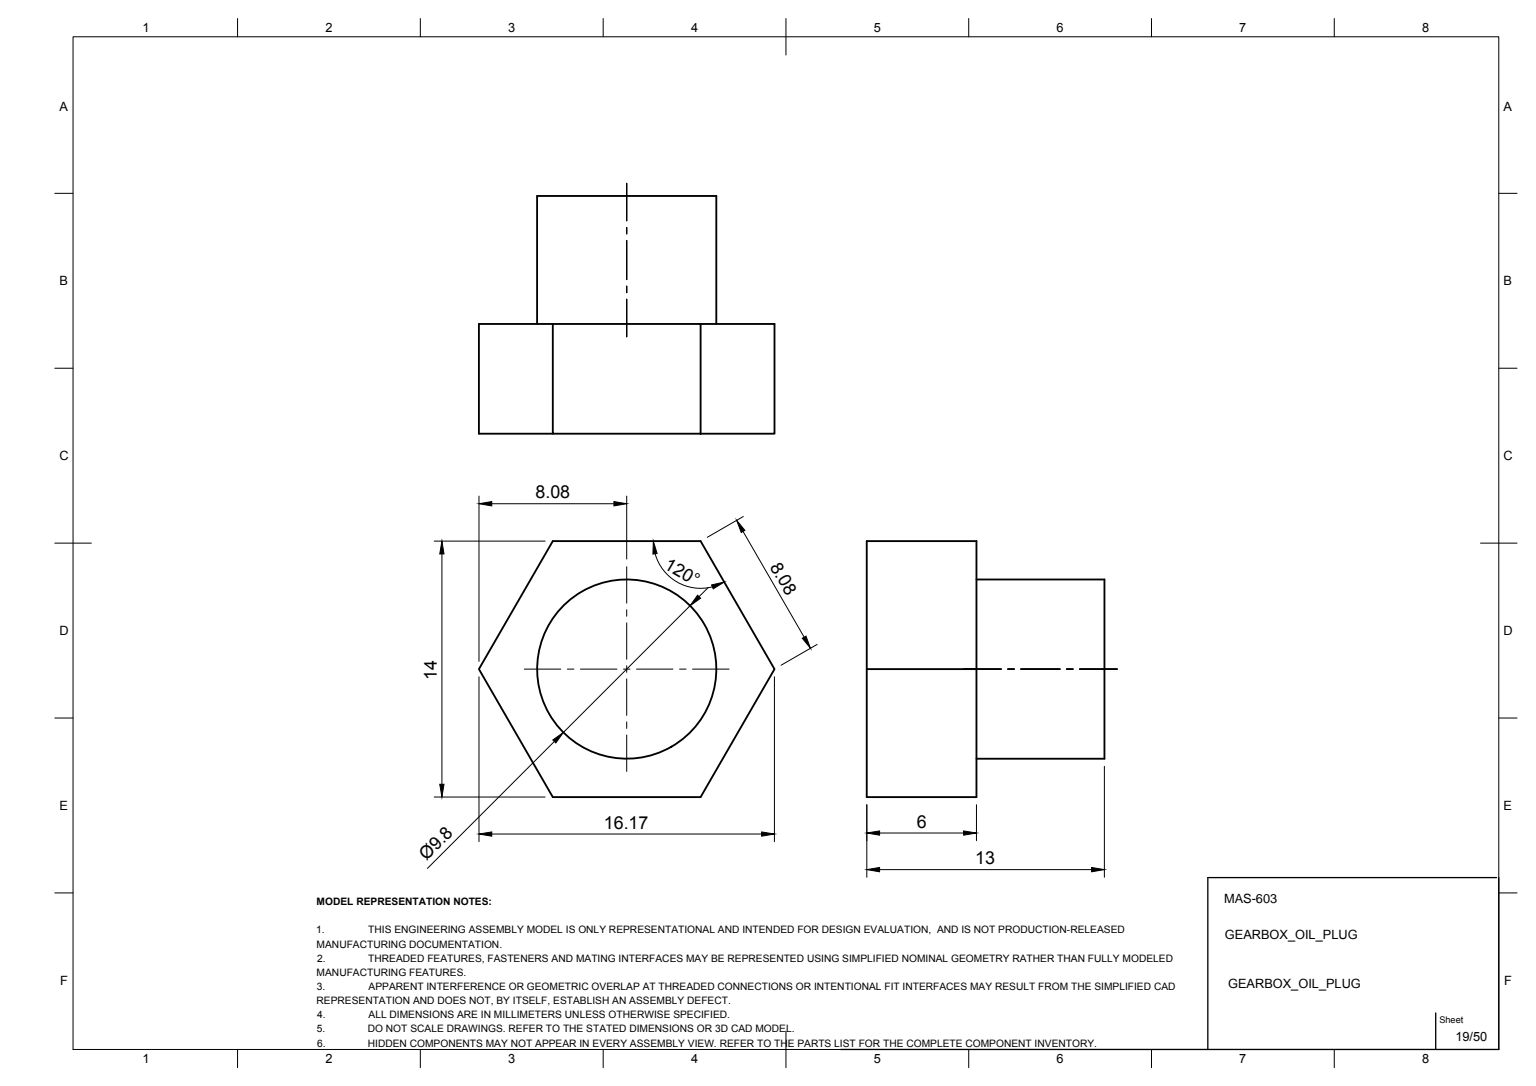
ISO-10303-21;
HEADER;
FILE_DESCRIPTION((''),'2;1');
FILE_NAME('GEARBOX_OIL_PLUG.step','2026-10-01T22:06:14-07:00',(''),(''),'','','');
FILE_SCHEMA (('AUTOMOTIVE_DESIGN { 1 0 10303 214 3 1 1 }'));
ENDSEC;
DATA;
#10=MECHANICAL_DESIGN_GEOMETRIC_PRESENTATION_REPRESENTATION('',(#991),#50440);
#901=SHAPE_REPRESENTATION_RELATIONSHIP('SRR','None',#50633,#946) ;
#946=ADVANCED_BREP_SHAPE_REPRESENTATION('',(#1046),#50402) ;
#991=STYLED_ITEM('',(#50887),#1046) ;
#1046=MANIFOLD_SOLID_BREP('GEARBOX_OIL_PLUG',#28658) ;
#1294=FACE_BOUND('',#4832,.T.) ;
#1979=PLANE('',#30398) ;
#1980=PLANE('',#30399) ;
#1981=PLANE('',#30400) ;
#1982=PLANE('',#30401) ;
#1983=PLANE('',#30402) ;
#1984=PLANE('',#30403) ;
#1985=PLANE('',#30404) ;
#1986=PLANE('',#30405) ;
#1987=PLANE('',#30406) ;
#3091=FACE_OUTER_BOUND('',#4827,.T.) ;
#3092=FACE_OUTER_BOUND('',#4828,.T.) ;
#3093=FACE_OUTER_BOUND('',#4829,.T.) ;
#3094=FACE_OUTER_BOUND('',#4830,.T.) ;
#3095=FACE_OUTER_BOUND('',#4831,.T.) ;
#3096=FACE_OUTER_BOUND('',#4833,.T.) ;
#3097=FACE_OUTER_BOUND('',#4834,.T.) ;
#3098=FACE_OUTER_BOUND('',#4835,.T.) ;
#3099=FACE_OUTER_BOUND('',#4836,.T.) ;
#3100=FACE_OUTER_BOUND('',#4837,.T.) ;
#4827=EDGE_LOOP('',(#22489,#22490,#22491,#22492)) ;
#4828=EDGE_LOOP('',(#22493)) ;
#4829=EDGE_LOOP('',(#22494,#22495,#22496,#22497)) ;
#4830=EDGE_LOOP('',(#22498,#22499,#22500,#22501)) ;
#4831=EDGE_LOOP('',(#22502,#22503,#22504,#22505,#22506,#22507)) ;
#4832=EDGE_LOOP('',(#22508)) ;
#4833=EDGE_LOOP('',(#22509,#22510,#22511,#22512)) ;
#4834=EDGE_LOOP('',(#22513,#22514,#22515,#22516)) ;
#4835=EDGE_LOOP('',(#22517,#22518,#22519,#22520)) ;
#4836=EDGE_LOOP('',(#22521,#22522,#22523,#22524)) ;
#4837=EDGE_LOOP('',(#22525,#22526,#22527,#22528,#22529,#22530)) ;
#7265=LINE('',#45416,#9737) ;
#7266=LINE('',#45422,#9738) ;
#7267=LINE('',#45424,#9739) ;
#7268=LINE('',#45426,#9740) ;
#7269=LINE('',#45427,#9741) ;
#7270=LINE('',#45431,#9742) ;
#7271=LINE('',#45433,#9743) ;
#7272=LINE('',#45435,#9744) ;
#7273=LINE('',#45436,#9745) ;
#7274=LINE('',#45439,#9746) ;
#7275=LINE('',#45440,#9747) ;
#7276=LINE('',#45442,#9748) ;
#7277=LINE('',#45443,#9749) ;
#7278=LINE('',#45446,#9750) ;
#7279=LINE('',#45447,#9751) ;
#7280=LINE('',#45450,#9752) ;
#7281=LINE('',#45451,#9753) ;
#7282=LINE('',#45453,#9754) ;
#7283=LINE('',#45455,#9755) ;
#9737=VECTOR('',#36284,0.49) ;
#9738=VECTOR('',#36291,1.) ;
#9739=VECTOR('',#36292,1.) ;
#9740=VECTOR('',#36293,1.) ;
#9741=VECTOR('',#36294,1.) ;
#9742=VECTOR('',#36297,1.) ;
#9743=VECTOR('',#36298,1.) ;
#9744=VECTOR('',#36299,1.) ;
#9745=VECTOR('',#36300,1.) ;
#9746=VECTOR('',#36303,1.) ;
#9747=VECTOR('',#36304,1.) ;
#9748=VECTOR('',#36305,1.) ;
#9749=VECTOR('',#36306,1.) ;
#9750=VECTOR('',#36309,1.) ;
#9751=VECTOR('',#36310,1.) ;
#9752=VECTOR('',#36313,1.) ;
#9753=VECTOR('',#36314,1.) ;
#9754=VECTOR('',#36317,1.) ;
#9755=VECTOR('',#36320,1.) ;
#11049=CIRCLE('',#30396,0.49) ;
#11050=CIRCLE('',#30397,0.49) ;
#13147=VERTEX_POINT('',#45413) ;
#13148=VERTEX_POINT('',#45415) ;
#13149=VERTEX_POINT('',#45420) ;
#13150=VERTEX_POINT('',#45421) ;
#13151=VERTEX_POINT('',#45423) ;
#13152=VERTEX_POINT('',#45425) ;
#13153=VERTEX_POINT('',#45429) ;
#13154=VERTEX_POINT('',#45430) ;
#13155=VERTEX_POINT('',#45432) ;
#13156=VERTEX_POINT('',#45434) ;
#13157=VERTEX_POINT('',#45438) ;
#13158=VERTEX_POINT('',#45441) ;
#13159=VERTEX_POINT('',#45445) ;
#13160=VERTEX_POINT('',#45449) ;
#16510=EDGE_CURVE('',#13147,#13147,#11049,.T.) ;
#16511=EDGE_CURVE('',#13147,#13148,#7265,.T.) ;
#16512=EDGE_CURVE('',#13148,#13148,#11050,.T.) ;
#16513=EDGE_CURVE('',#13149,#13150,#7266,.T.) ;
#16514=EDGE_CURVE('',#13149,#13151,#7267,.T.) ;
#16515=EDGE_CURVE('',#13152,#13151,#7268,.T.) ;
#16516=EDGE_CURVE('',#13152,#13150,#7269,.T.) ;
#16517=EDGE_CURVE('',#13153,#13154,#7270,.T.) ;
#16518=EDGE_CURVE('',#13153,#13155,#7271,.T.) ;
#16519=EDGE_CURVE('',#13156,#13155,#7272,.T.) ;
#16520=EDGE_CURVE('',#13156,#13154,#7273,.T.) ;
#16521=EDGE_CURVE('',#13157,#13149,#7274,.T.) ;
#16522=EDGE_CURVE('',#13155,#13157,#7275,.T.) ;
#16523=EDGE_CURVE('',#13158,#13153,#7276,.T.) ;
#16524=EDGE_CURVE('',#13151,#13158,#7277,.T.) ;
#16525=EDGE_CURVE('',#13157,#13159,#7278,.T.) ;
#16526=EDGE_CURVE('',#13150,#13159,#7279,.T.) ;
#16527=EDGE_CURVE('',#13158,#13160,#7280,.T.) ;
#16528=EDGE_CURVE('',#13154,#13160,#7281,.T.) ;
#16529=EDGE_CURVE('',#13159,#13156,#7282,.T.) ;
#16530=EDGE_CURVE('',#13160,#13152,#7283,.T.) ;
#22489=ORIENTED_EDGE('',*,*,#16510,.F.) ;
#22490=ORIENTED_EDGE('',*,*,#16511,.T.) ;
#22491=ORIENTED_EDGE('',*,*,#16512,.F.) ;
#22492=ORIENTED_EDGE('',*,*,#16511,.F.) ;
#22493=ORIENTED_EDGE('',*,*,#16512,.T.) ;
#22494=ORIENTED_EDGE('',*,*,#16513,.F.) ;
#22495=ORIENTED_EDGE('',*,*,#16514,.T.) ;
#22496=ORIENTED_EDGE('',*,*,#16515,.F.) ;
#22497=ORIENTED_EDGE('',*,*,#16516,.T.) ;
#22498=ORIENTED_EDGE('',*,*,#16517,.F.) ;
#22499=ORIENTED_EDGE('',*,*,#16518,.T.) ;
#22500=ORIENTED_EDGE('',*,*,#16519,.F.) ;
#22501=ORIENTED_EDGE('',*,*,#16520,.T.) ;
#22502=ORIENTED_EDGE('',*,*,#16514,.F.) ;
#22503=ORIENTED_EDGE('',*,*,#16521,.F.) ;
#22504=ORIENTED_EDGE('',*,*,#16522,.F.) ;
#22505=ORIENTED_EDGE('',*,*,#16518,.F.) ;
#22506=ORIENTED_EDGE('',*,*,#16523,.F.) ;
#22507=ORIENTED_EDGE('',*,*,#16524,.F.) ;
#22508=ORIENTED_EDGE('',*,*,#16510,.T.) ;
#22509=ORIENTED_EDGE('',*,*,#16525,.F.) ;
#22510=ORIENTED_EDGE('',*,*,#16521,.T.) ;
#22511=ORIENTED_EDGE('',*,*,#16513,.T.) ;
#22512=ORIENTED_EDGE('',*,*,#16526,.T.) ;
#22513=ORIENTED_EDGE('',*,*,#16527,.F.) ;
#22514=ORIENTED_EDGE('',*,*,#16523,.T.) ;
#22515=ORIENTED_EDGE('',*,*,#16517,.T.) ;
#22516=ORIENTED_EDGE('',*,*,#16528,.T.) ;
#22517=ORIENTED_EDGE('',*,*,#16519,.T.) ;
#22518=ORIENTED_EDGE('',*,*,#16522,.T.) ;
#22519=ORIENTED_EDGE('',*,*,#16525,.T.) ;
#22520=ORIENTED_EDGE('',*,*,#16529,.T.) ;
#22521=ORIENTED_EDGE('',*,*,#16527,.T.) ;
#22522=ORIENTED_EDGE('',*,*,#16530,.T.) ;
#22523=ORIENTED_EDGE('',*,*,#16515,.T.) ;
#22524=ORIENTED_EDGE('',*,*,#16524,.T.) ;
#22525=ORIENTED_EDGE('',*,*,#16516,.F.) ;
#22526=ORIENTED_EDGE('',*,*,#16530,.F.) ;
#22527=ORIENTED_EDGE('',*,*,#16528,.F.) ;
#22528=ORIENTED_EDGE('',*,*,#16520,.F.) ;
#22529=ORIENTED_EDGE('',*,*,#16529,.F.) ;
#22530=ORIENTED_EDGE('',*,*,#16526,.F.) ;
#26801=CYLINDRICAL_SURFACE('',#30395,0.49) ;
#27826=ADVANCED_FACE('',(#3091),#26801,.T.) ;
#27827=ADVANCED_FACE('',(#3092),#1979,.T.) ;
#27828=ADVANCED_FACE('',(#3093),#1980,.F.) ;
#27829=ADVANCED_FACE('',(#3094),#1981,.F.) ;
#27830=ADVANCED_FACE('',(#3095,#1294),#1982,.T.) ;
#27831=ADVANCED_FACE('',(#3096),#1983,.F.) ;
#27832=ADVANCED_FACE('',(#3097),#1984,.F.) ;
#27833=ADVANCED_FACE('',(#3098),#1985,.F.) ;
#27834=ADVANCED_FACE('',(#3099),#1986,.F.) ;
#27835=ADVANCED_FACE('',(#3100),#1987,.T.) ;
#28658=CLOSED_SHELL('',(#27826,#27827,#27828,#27829,#27830,#27831,#27832,
#27833,#27834,#27835)) ;
#30394=AXIS2_PLACEMENT_3D('',#45411,#36278,#36279) ;
#30395=AXIS2_PLACEMENT_3D('',#45412,#36280,#36281) ;
#30396=AXIS2_PLACEMENT_3D('',#45414,#36282,#36283) ;
#30397=AXIS2_PLACEMENT_3D('',#45417,#36285,#36286) ;
#30398=AXIS2_PLACEMENT_3D('',#45418,#36287,#36288) ;
#30399=AXIS2_PLACEMENT_3D('',#45419,#36289,#36290) ;
#30400=AXIS2_PLACEMENT_3D('',#45428,#36295,#36296) ;
#30401=AXIS2_PLACEMENT_3D('',#45437,#36301,#36302) ;
#30402=AXIS2_PLACEMENT_3D('',#45444,#36307,#36308) ;
#30403=AXIS2_PLACEMENT_3D('',#45448,#36311,#36312) ;
#30404=AXIS2_PLACEMENT_3D('',#45452,#36315,#36316) ;
#30405=AXIS2_PLACEMENT_3D('',#45454,#36318,#36319) ;
#30406=AXIS2_PLACEMENT_3D('',#45456,#36321,#36322) ;
#36278=DIRECTION('axis',(0.,0.,1.)) ;
#36279=DIRECTION('refdir',(1.,0.,0.)) ;
#36280=DIRECTION('center_axis',(1.,0.,0.)) ;
#36281=DIRECTION('ref_axis',(0.,0.,-1.)) ;
#36282=DIRECTION('center_axis',(1.,0.,0.)) ;
#36283=DIRECTION('ref_axis',(0.,0.,-1.)) ;
#36284=DIRECTION('',(-1.,0.,0.)) ;
#36285=DIRECTION('center_axis',(-1.,0.,0.)) ;
#36286=DIRECTION('ref_axis',(0.,0.,-1.)) ;
#36287=DIRECTION('center_axis',(-1.,0.,0.)) ;
#36288=DIRECTION('ref_axis',(0.,0.,1.)) ;
#36289=DIRECTION('center_axis',(0.,-0.866025403784439,-0.5)) ;
#36290=DIRECTION('ref_axis',(0.,0.5,-0.866025403784439)) ;
#36291=DIRECTION('',(1.,0.,0.)) ;
#36292=DIRECTION('',(0.,-0.5,0.866025403784439)) ;
#36293=DIRECTION('',(-1.,0.,0.)) ;
#36294=DIRECTION('',(0.,0.5,-0.866025403784439)) ;
#36295=DIRECTION('center_axis',(0.,0.866025403784439,0.5)) ;
#36296=DIRECTION('ref_axis',(0.,-0.5,0.866025403784439)) ;
#36297=DIRECTION('',(1.,0.,0.)) ;
#36298=DIRECTION('',(0.,0.5,-0.866025403784439)) ;
#36299=DIRECTION('',(-1.,0.,0.)) ;
#36300=DIRECTION('',(0.,-0.5,0.866025403784439)) ;
#36301=DIRECTION('center_axis',(-1.,0.,0.)) ;
#36302=DIRECTION('ref_axis',(0.,0.,1.)) ;
#36303=DIRECTION('',(0.,0.5,0.866025403784439)) ;
#36304=DIRECTION('',(0.,1.,0.)) ;
#36305=DIRECTION('',(0.,-0.5,-0.866025403784439)) ;
#36306=DIRECTION('',(0.,-1.,0.)) ;
#36307=DIRECTION('center_axis',(0.,-0.866025403784439,0.5)) ;
#36308=DIRECTION('ref_axis',(0.,-0.5,-0.866025403784439)) ;
#36309=DIRECTION('',(1.,0.,0.)) ;
#36310=DIRECTION('',(0.,-0.5,-0.866025403784439)) ;
#36311=DIRECTION('center_axis',(0.,0.866025403784439,-0.5)) ;
#36312=DIRECTION('ref_axis',(0.,0.5,0.866025403784439)) ;
#36313=DIRECTION('',(1.,0.,0.)) ;
#36314=DIRECTION('',(0.,0.5,0.866025403784439)) ;
#36315=DIRECTION('center_axis',(0.,0.,1.)) ;
#36316=DIRECTION('ref_axis',(0.,-1.,0.)) ;
#36317=DIRECTION('',(0.,-1.,0.)) ;
#36318=DIRECTION('center_axis',(0.,0.,-1.)) ;
#36319=DIRECTION('ref_axis',(0.,1.,0.)) ;
#36320=DIRECTION('',(0.,1.,0.)) ;
#36321=DIRECTION('center_axis',(1.,0.,0.)) ;
#36322=DIRECTION('ref_axis',(0.,0.,-1.)) ;
#45411=CARTESIAN_POINT('',(0.,0.,0.)) ;
#45412=CARTESIAN_POINT('Origin',(11.45,7.,38.)) ;
#45413=CARTESIAN_POINT('',(11.8,7.,38.49)) ;
#45414=CARTESIAN_POINT('Origin',(11.8,7.,38.)) ;
#45415=CARTESIAN_POINT('',(11.1,7.,38.49)) ;
#45416=CARTESIAN_POINT('',(11.45,7.,38.49)) ;
#45417=CARTESIAN_POINT('Origin',(11.1,7.,38.)) ;
#45418=CARTESIAN_POINT('Origin',(11.1,7.,38.)) ;
#45419=CARTESIAN_POINT('Origin',(12.1,7.60621778264911,38.35)) ;
#45420=CARTESIAN_POINT('',(11.8,7.80829037686548,38.)) ;
#45421=CARTESIAN_POINT('',(12.4,7.80829037686548,38.)) ;
#45422=CARTESIAN_POINT('',(12.1,7.80829037686548,38.)) ;
#45423=CARTESIAN_POINT('',(11.8,7.40414518843273,38.7)) ;
#45424=CARTESIAN_POINT('',(11.8,7.60621778264911,38.35)) ;
#45425=CARTESIAN_POINT('',(12.4,7.40414518843273,38.7)) ;
#45426=CARTESIAN_POINT('',(12.1,7.40414518843273,38.7)) ;
#45427=CARTESIAN_POINT('',(12.4,7.60621778264911,38.35)) ;
#45428=CARTESIAN_POINT('Origin',(12.1,6.39378221735089,37.65)) ;
#45429=CARTESIAN_POINT('',(11.8,6.19170962313452,38.)) ;
#45430=CARTESIAN_POINT('',(12.4,6.19170962313452,38.)) ;
#45431=CARTESIAN_POINT('',(12.1,6.19170962313452,38.)) ;
#45432=CARTESIAN_POINT('',(11.8,6.59585481156727,37.3)) ;
#45433=CARTESIAN_POINT('',(11.8,6.39378221735089,37.65)) ;
#45434=CARTESIAN_POINT('',(12.4,6.59585481156727,37.3)) ;
#45435=CARTESIAN_POINT('',(12.1,6.59585481156727,37.3)) ;
#45436=CARTESIAN_POINT('',(12.4,6.39378221735089,37.65)) ;
#45437=CARTESIAN_POINT('Origin',(11.8,7.,38.)) ;
#45438=CARTESIAN_POINT('',(11.8,7.40414518843273,37.3)) ;
#45439=CARTESIAN_POINT('',(11.8,7.60621778264911,37.65)) ;
#45440=CARTESIAN_POINT('',(11.8,7.,37.3)) ;
#45441=CARTESIAN_POINT('',(11.8,6.59585481156727,38.7)) ;
#45442=CARTESIAN_POINT('',(11.8,6.39378221735089,38.35)) ;
#45443=CARTESIAN_POINT('',(11.8,7.,38.7)) ;
#45444=CARTESIAN_POINT('Origin',(12.1,7.60621778264911,37.65)) ;
#45445=CARTESIAN_POINT('',(12.4,7.40414518843273,37.3)) ;
#45446=CARTESIAN_POINT('',(12.1,7.40414518843273,37.3)) ;
#45447=CARTESIAN_POINT('',(12.4,7.60621778264911,37.65)) ;
#45448=CARTESIAN_POINT('Origin',(12.1,6.39378221735089,38.35)) ;
#45449=CARTESIAN_POINT('',(12.4,6.59585481156727,38.7)) ;
#45450=CARTESIAN_POINT('',(12.1,6.59585481156727,38.7)) ;
#45451=CARTESIAN_POINT('',(12.4,6.39378221735089,38.35)) ;
#45452=CARTESIAN_POINT('Origin',(12.1,7.,37.3)) ;
#45453=CARTESIAN_POINT('',(12.4,7.,37.3)) ;
#45454=CARTESIAN_POINT('Origin',(12.1,7.,38.7)) ;
#45455=CARTESIAN_POINT('',(12.4,7.,38.7)) ;
#45456=CARTESIAN_POINT('Origin',(12.4,7.,38.)) ;
#50349=UNCERTAINTY_MEASURE_WITH_UNIT(LENGTH_MEASURE(0.001),#50441,
'DISTANCE_ACCURACY_VALUE',
'Maximum model space distance between geometric entities at asserted c
onnectivities') ;
#50387=UNCERTAINTY_MEASURE_WITH_UNIT(LENGTH_MEASURE(0.001),#50441,
'DISTANCE_ACCURACY_VALUE',
'Maximum model space distance between geometric entities at asserted c
onnectivities') ;
#50402=(
GEOMETRIC_REPRESENTATION_CONTEXT(3)
GLOBAL_UNCERTAINTY_ASSIGNED_CONTEXT((#50349))
GLOBAL_UNIT_ASSIGNED_CONTEXT((#50441,#50443,#50444))
REPRESENTATION_CONTEXT('','3D')
) ;
#50440=(
GEOMETRIC_REPRESENTATION_CONTEXT(3)
GLOBAL_UNCERTAINTY_ASSIGNED_CONTEXT((#50387))
GLOBAL_UNIT_ASSIGNED_CONTEXT((#50441,#50443,#50444))
REPRESENTATION_CONTEXT('','3D')
) ;
#50441=(
LENGTH_UNIT()
NAMED_UNIT(*)
SI_UNIT(.CENTI.,.METRE.)
) ;
#50443=(
NAMED_UNIT(*)
PLANE_ANGLE_UNIT()
SI_UNIT($,.RADIAN.)
) ;
#50444=(
NAMED_UNIT(*)
SI_UNIT($,.STERADIAN.)
SOLID_ANGLE_UNIT()
) ;
#50459=SHAPE_DEFINITION_REPRESENTATION(#50525,#50633) ;
#50525=PRODUCT_DEFINITION_SHAPE('',$,#50686) ;
#50633=SHAPE_REPRESENTATION('',(#30394),#50402) ;
#50671=PRODUCT_DEFINITION_CONTEXT('part definition',#50829,'design') ;
#50686=PRODUCT_DEFINITION('GEARBOX_OIL_PLUG','GEARBOX_OIL_PLUG',
#50738,#50671) ;
#50738=PRODUCT_DEFINITION_FORMATION('',$,#50845) ;
#50829=APPLICATION_CONTEXT(
'Core Data for Automotive Mechanical Design Process') ;
#50830=PRODUCT_CONTEXT('part definition',#50829,'mechanical') ;
#50845=PRODUCT('GEARBOX_OIL_PLUG','GEARBOX_OIL_PLUG',$,(#50830)) ;
#50887=PRESENTATION_STYLE_ASSIGNMENT((#50894)) ;
#50894=SURFACE_STYLE_USAGE(.BOTH.,#50901) ;
#50901=SURFACE_SIDE_STYLE('',(#50908)) ;
#50908=SURFACE_STYLE_FILL_AREA(#50915) ;
#50915=FILL_AREA_STYLE('Brass - Polished',(#50922)) ;
#50922=FILL_AREA_STYLE_COLOUR('Brass - Polished',#50929) ;
#50929=COLOUR_RGB('Brass - Polished', 0.66274510, 0.83137255, 0.94901961) ;
ENDSEC;
END-ISO-10303-21;
